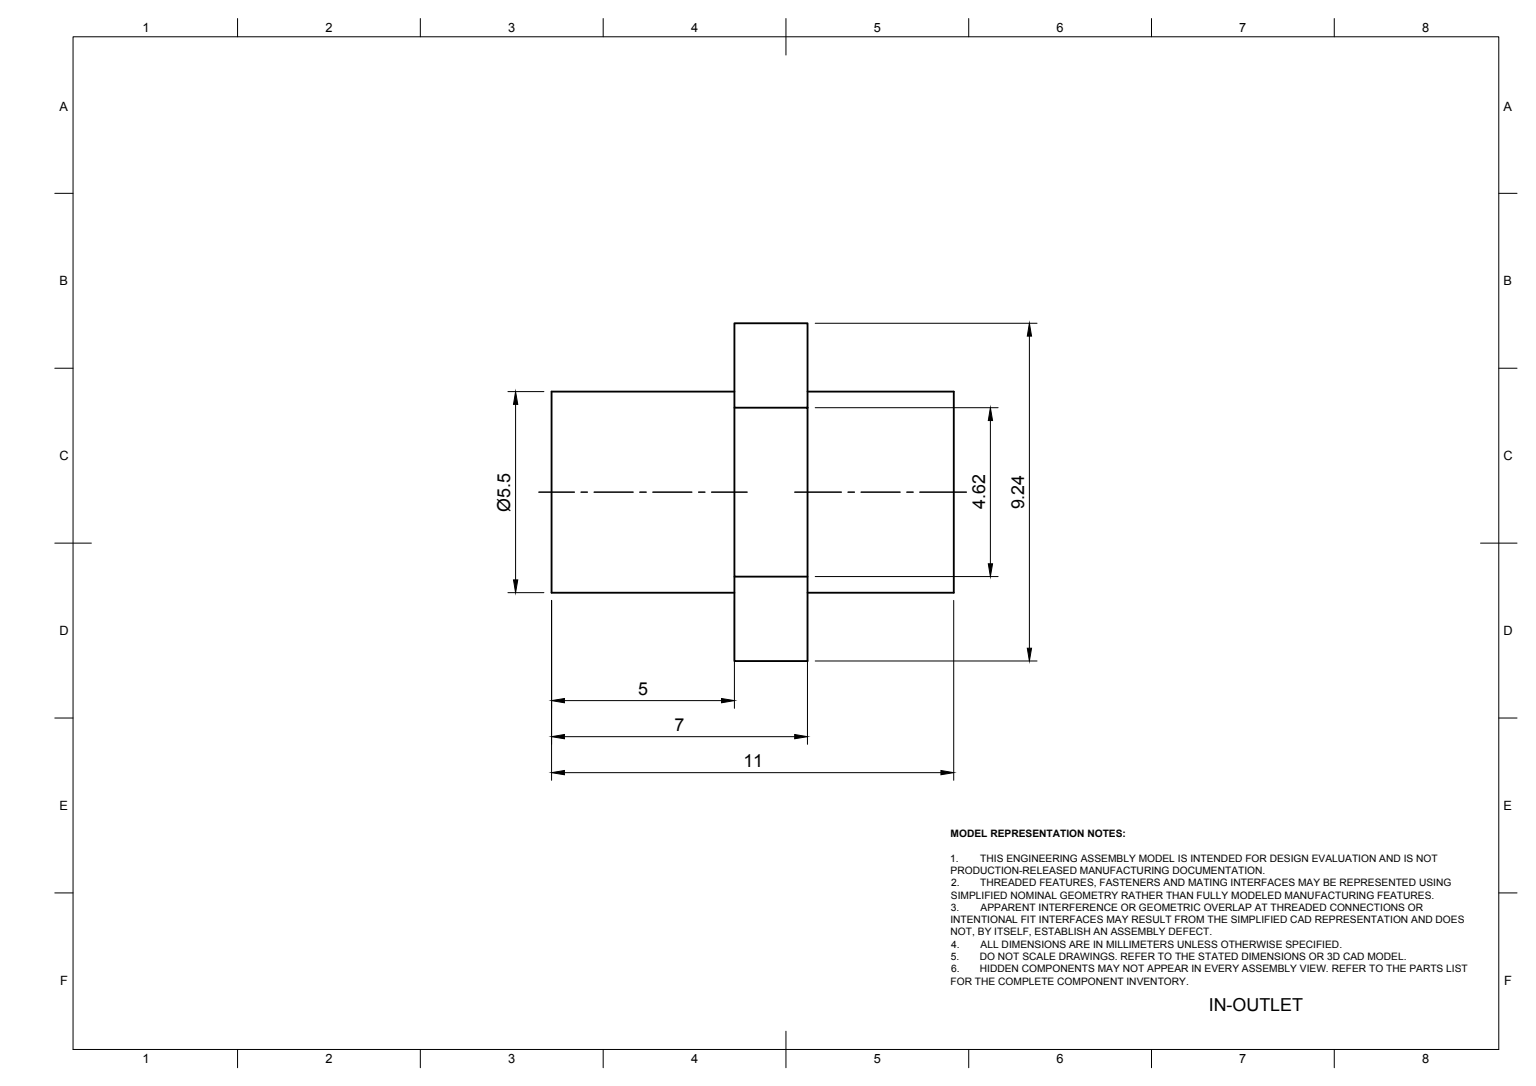
ISO-10303-21;
HEADER;
/* Generated by software containing ST-Developer
 * from STEP Tools, Inc. (www.steptools.com) 
 */

FILE_DESCRIPTION(
/* description */ (''),
/* implementation_level */ '2;1');

FILE_NAME(
/* name */ 'IN-OUTLET.step',
/* time_stamp */ '2026-10-06T01:16:10-07:00',
/* author */ (''),
/* organization */ (''),
/* preprocessor_version */ 'ST-DEVELOPER v20.2',
/* originating_system */ 'Autodesk Translation Framework v15.15.0.0',
/* authorisation */ '');

FILE_SCHEMA (('AUTOMOTIVE_DESIGN { 1 0 10303 214 3 1 1 }'));
ENDSEC;

DATA;
#10=MECHANICAL_DESIGN_GEOMETRIC_PRESENTATION_REPRESENTATION('',(#303,#304,#305),#17113);
#225=OPEN_SHELL('',(#5821,#5822));
#226=OPEN_SHELL('',(#5823,#5824));
#243=SHELL_BASED_SURFACE_MODEL('Body2',(#225));
#244=SHELL_BASED_SURFACE_MODEL('Body3',(#226));
#267=SHAPE_REPRESENTATION_RELATIONSHIP('SRR','None',#17189,#283);
#283=ADVANCED_BREP_SHAPE_REPRESENTATION('',(#333),#17096);
#303=STYLED_ITEM('',(#17298),#333);
#304=STYLED_ITEM('',(#17298),#243);
#305=STYLED_ITEM('',(#17298),#244);
#333=MANIFOLD_SOLID_BREP('Body1',#6019);
#410=CYLINDRICAL_SURFACE('',#6534,2.75);
#411=CYLINDRICAL_SURFACE('',#6536,2.75);
#412=CYLINDRICAL_SURFACE('',#6540,1.75);
#413=CYLINDRICAL_SURFACE('',#6543,2.475);
#414=CYLINDRICAL_SURFACE('',#6548,2.475);
#545=FACE_BOUND('',#1562,.T.);
#546=FACE_BOUND('',#1570,.T.);
#547=FACE_BOUND('',#1574,.T.);
#548=FACE_BOUND('',#1577,.T.);
#549=FACE_BOUND('',#1580,.T.);
#550=FACE_BOUND('',#1583,.T.);
#796=CIRCLE('',#6525,2.75);
#797=CIRCLE('',#6533,2.75);
#798=CIRCLE('',#6535,2.75);
#799=CIRCLE('',#6537,2.75);
#800=CIRCLE('',#6539,1.75);
#801=CIRCLE('',#6541,1.75);
#802=CIRCLE('',#6544,2.475);
#803=CIRCLE('',#6545,2.475);
#804=CIRCLE('',#6547,2.75);
#805=CIRCLE('',#6549,2.475);
#806=CIRCLE('',#6550,2.475);
#807=CIRCLE('',#6552,2.75);
#1160=FACE_OUTER_BOUND('',#1561,.T.);
#1161=FACE_OUTER_BOUND('',#1563,.T.);
#1162=FACE_OUTER_BOUND('',#1564,.T.);
#1163=FACE_OUTER_BOUND('',#1565,.T.);
#1164=FACE_OUTER_BOUND('',#1566,.T.);
#1165=FACE_OUTER_BOUND('',#1567,.T.);
#1166=FACE_OUTER_BOUND('',#1568,.T.);
#1167=FACE_OUTER_BOUND('',#1569,.T.);
#1168=FACE_OUTER_BOUND('',#1571,.T.);
#1169=FACE_OUTER_BOUND('',#1572,.T.);
#1170=FACE_OUTER_BOUND('',#1573,.T.);
#1171=FACE_OUTER_BOUND('',#1575,.T.);
#1172=FACE_OUTER_BOUND('',#1576,.T.);
#1173=FACE_OUTER_BOUND('',#1578,.T.);
#1174=FACE_OUTER_BOUND('',#1579,.T.);
#1175=FACE_OUTER_BOUND('',#1581,.T.);
#1176=FACE_OUTER_BOUND('',#1582,.T.);
#1561=EDGE_LOOP('',(#4622,#4623,#4624,#4625,#4626,#4627));
#1562=EDGE_LOOP('',(#4628));
#1563=EDGE_LOOP('',(#4629,#4630,#4631,#4632));
#1564=EDGE_LOOP('',(#4633,#4634,#4635,#4636));
#1565=EDGE_LOOP('',(#4637,#4638,#4639,#4640));
#1566=EDGE_LOOP('',(#4641,#4642,#4643,#4644));
#1567=EDGE_LOOP('',(#4645,#4646,#4647,#4648));
#1568=EDGE_LOOP('',(#4649,#4650,#4651,#4652));
#1569=EDGE_LOOP('',(#4653,#4654,#4655,#4656,#4657,#4658));
#1570=EDGE_LOOP('',(#4659));
#1571=EDGE_LOOP('',(#4660,#4661,#4662,#4663));
#1572=EDGE_LOOP('',(#4664,#4665,#4666,#4667));
#1573=EDGE_LOOP('',(#4668));
#1574=EDGE_LOOP('',(#4669));
#1575=EDGE_LOOP('',(#4670,#4671,#4672,#4673));
#1576=EDGE_LOOP('',(#4674));
#1577=EDGE_LOOP('',(#4675));
#1578=EDGE_LOOP('',(#4676,#4677,#4678,#4679));
#1579=EDGE_LOOP('',(#4680));
#1580=EDGE_LOOP('',(#4681));
#1581=EDGE_LOOP('',(#4682,#4683,#4684,#4685));
#1582=EDGE_LOOP('',(#4686));
#1583=EDGE_LOOP('',(#4687));
#2031=LINE('',#10370,#2392);
#2032=LINE('',#10372,#2393);
#2033=LINE('',#10374,#2394);
#2034=LINE('',#10376,#2395);
#2035=LINE('',#10378,#2396);
#2036=LINE('',#10379,#2397);
#2037=LINE('',#10384,#2398);
#2038=LINE('',#10386,#2399);
#2039=LINE('',#10387,#2400);
#2040=LINE('',#10390,#2401);
#2041=LINE('',#10391,#2402);
#2042=LINE('',#10394,#2403);
#2043=LINE('',#10395,#2404);
#2044=LINE('',#10398,#2405);
#2045=LINE('',#10399,#2406);
#2046=LINE('',#10402,#2407);
#2047=LINE('',#10403,#2408);
#2048=LINE('',#10405,#2409);
#2049=LINE('',#10411,#2410);
#2050=LINE('',#10416,#2411);
#2051=LINE('',#10422,#2412);
#2052=LINE('',#10429,#2413);
#2053=LINE('',#10438,#2414);
#2392=VECTOR('',#7781,4.618802153517);
#2393=VECTOR('',#7782,4.61880215351685);
#2394=VECTOR('',#7783,4.61880215351685);
#2395=VECTOR('',#7784,4.618802153517);
#2396=VECTOR('',#7785,4.61880215351685);
#2397=VECTOR('',#7786,4.61880215351685);
#2398=VECTOR('',#7791,2.);
#2399=VECTOR('',#7792,4.618802153517);
#2400=VECTOR('',#7793,2.);
#2401=VECTOR('',#7796,4.61880215351685);
#2402=VECTOR('',#7797,2.);
#2403=VECTOR('',#7800,4.61880215351685);
#2404=VECTOR('',#7801,2.);
#2405=VECTOR('',#7804,4.618802153517);
#2406=VECTOR('',#7805,2.);
#2407=VECTOR('',#7808,4.61880215351685);
#2408=VECTOR('',#7809,2.);
#2409=VECTOR('',#7812,4.61880215351685);
#2410=VECTOR('',#7819,2.75);
#2411=VECTOR('',#7826,2.75);
#2412=VECTOR('',#7833,1.75);
#2413=VECTOR('',#7842,2.475);
#2414=VECTOR('',#7853,2.475);
#2800=VERTEX_POINT('',#10368);
#2801=VERTEX_POINT('',#10369);
#2802=VERTEX_POINT('',#10371);
#2803=VERTEX_POINT('',#10373);
#2804=VERTEX_POINT('',#10375);
#2805=VERTEX_POINT('',#10377);
#2806=VERTEX_POINT('',#10380);
#2807=VERTEX_POINT('',#10383);
#2808=VERTEX_POINT('',#10385);
#2809=VERTEX_POINT('',#10389);
#2810=VERTEX_POINT('',#10393);
#2811=VERTEX_POINT('',#10397);
#2812=VERTEX_POINT('',#10401);
#2813=VERTEX_POINT('',#10407);
#2814=VERTEX_POINT('',#10410);
#2815=VERTEX_POINT('',#10414);
#2816=VERTEX_POINT('',#10418);
#2817=VERTEX_POINT('',#10421);
#2818=VERTEX_POINT('',#10426);
#2819=VERTEX_POINT('',#10428);
#2820=VERTEX_POINT('',#10432);
#2821=VERTEX_POINT('',#10435);
#2822=VERTEX_POINT('',#10437);
#2823=VERTEX_POINT('',#10441);
#3461=EDGE_CURVE('',#2800,#2801,#2031,.T.);
#3462=EDGE_CURVE('',#2802,#2800,#2032,.T.);
#3463=EDGE_CURVE('',#2803,#2802,#2033,.T.);
#3464=EDGE_CURVE('',#2804,#2803,#2034,.T.);
#3465=EDGE_CURVE('',#2805,#2804,#2035,.T.);
#3466=EDGE_CURVE('',#2801,#2805,#2036,.T.);
#3467=EDGE_CURVE('',#2806,#2806,#796,.T.);
#3468=EDGE_CURVE('',#2801,#2807,#2037,.T.);
#3469=EDGE_CURVE('',#2808,#2807,#2038,.T.);
#3470=EDGE_CURVE('',#2800,#2808,#2039,.T.);
#3471=EDGE_CURVE('',#2809,#2808,#2040,.T.);
#3472=EDGE_CURVE('',#2802,#2809,#2041,.T.);
#3473=EDGE_CURVE('',#2810,#2809,#2042,.T.);
#3474=EDGE_CURVE('',#2803,#2810,#2043,.T.);
#3475=EDGE_CURVE('',#2811,#2810,#2044,.T.);
#3476=EDGE_CURVE('',#2804,#2811,#2045,.T.);
#3477=EDGE_CURVE('',#2812,#2811,#2046,.T.);
#3478=EDGE_CURVE('',#2805,#2812,#2047,.T.);
#3479=EDGE_CURVE('',#2807,#2812,#2048,.T.);
#3480=EDGE_CURVE('',#2813,#2813,#797,.T.);
#3481=EDGE_CURVE('',#2806,#2814,#2049,.T.);
#3482=EDGE_CURVE('',#2814,#2814,#798,.T.);
#3483=EDGE_CURVE('',#2815,#2815,#799,.T.);
#3484=EDGE_CURVE('',#2815,#2813,#2050,.T.);
#3485=EDGE_CURVE('',#2816,#2816,#800,.T.);
#3486=EDGE_CURVE('',#2816,#2817,#2051,.T.);
#3487=EDGE_CURVE('',#2817,#2817,#801,.T.);
#3488=EDGE_CURVE('',#2818,#2818,#802,.T.);
#3489=EDGE_CURVE('',#2818,#2819,#2052,.T.);
#3490=EDGE_CURVE('',#2819,#2819,#803,.T.);
#3491=EDGE_CURVE('',#2820,#2820,#804,.T.);
#3492=EDGE_CURVE('',#2821,#2821,#805,.T.);
#3493=EDGE_CURVE('',#2821,#2822,#2053,.T.);
#3494=EDGE_CURVE('',#2822,#2822,#806,.T.);
#3495=EDGE_CURVE('',#2823,#2823,#807,.T.);
#4622=ORIENTED_EDGE('',*,*,#3461,.F.);
#4623=ORIENTED_EDGE('',*,*,#3462,.F.);
#4624=ORIENTED_EDGE('',*,*,#3463,.F.);
#4625=ORIENTED_EDGE('',*,*,#3464,.F.);
#4626=ORIENTED_EDGE('',*,*,#3465,.F.);
#4627=ORIENTED_EDGE('',*,*,#3466,.F.);
#4628=ORIENTED_EDGE('',*,*,#3467,.T.);
#4629=ORIENTED_EDGE('',*,*,#3461,.T.);
#4630=ORIENTED_EDGE('',*,*,#3468,.T.);
#4631=ORIENTED_EDGE('',*,*,#3469,.F.);
#4632=ORIENTED_EDGE('',*,*,#3470,.F.);
#4633=ORIENTED_EDGE('',*,*,#3462,.T.);
#4634=ORIENTED_EDGE('',*,*,#3470,.T.);
#4635=ORIENTED_EDGE('',*,*,#3471,.F.);
#4636=ORIENTED_EDGE('',*,*,#3472,.F.);
#4637=ORIENTED_EDGE('',*,*,#3463,.T.);
#4638=ORIENTED_EDGE('',*,*,#3472,.T.);
#4639=ORIENTED_EDGE('',*,*,#3473,.F.);
#4640=ORIENTED_EDGE('',*,*,#3474,.F.);
#4641=ORIENTED_EDGE('',*,*,#3464,.T.);
#4642=ORIENTED_EDGE('',*,*,#3474,.T.);
#4643=ORIENTED_EDGE('',*,*,#3475,.F.);
#4644=ORIENTED_EDGE('',*,*,#3476,.F.);
#4645=ORIENTED_EDGE('',*,*,#3465,.T.);
#4646=ORIENTED_EDGE('',*,*,#3476,.T.);
#4647=ORIENTED_EDGE('',*,*,#3477,.F.);
#4648=ORIENTED_EDGE('',*,*,#3478,.F.);
#4649=ORIENTED_EDGE('',*,*,#3466,.T.);
#4650=ORIENTED_EDGE('',*,*,#3478,.T.);
#4651=ORIENTED_EDGE('',*,*,#3479,.F.);
#4652=ORIENTED_EDGE('',*,*,#3468,.F.);
#4653=ORIENTED_EDGE('',*,*,#3469,.T.);
#4654=ORIENTED_EDGE('',*,*,#3479,.T.);
#4655=ORIENTED_EDGE('',*,*,#3477,.T.);
#4656=ORIENTED_EDGE('',*,*,#3475,.T.);
#4657=ORIENTED_EDGE('',*,*,#3473,.T.);
#4658=ORIENTED_EDGE('',*,*,#3471,.T.);
#4659=ORIENTED_EDGE('',*,*,#3480,.F.);
#4660=ORIENTED_EDGE('',*,*,#3467,.F.);
#4661=ORIENTED_EDGE('',*,*,#3481,.T.);
#4662=ORIENTED_EDGE('',*,*,#3482,.T.);
#4663=ORIENTED_EDGE('',*,*,#3481,.F.);
#4664=ORIENTED_EDGE('',*,*,#3483,.F.);
#4665=ORIENTED_EDGE('',*,*,#3484,.T.);
#4666=ORIENTED_EDGE('',*,*,#3480,.T.);
#4667=ORIENTED_EDGE('',*,*,#3484,.F.);
#4668=ORIENTED_EDGE('',*,*,#3482,.F.);
#4669=ORIENTED_EDGE('',*,*,#3485,.T.);
#4670=ORIENTED_EDGE('',*,*,#3485,.F.);
#4671=ORIENTED_EDGE('',*,*,#3486,.T.);
#4672=ORIENTED_EDGE('',*,*,#3487,.T.);
#4673=ORIENTED_EDGE('',*,*,#3486,.F.);
#4674=ORIENTED_EDGE('',*,*,#3483,.T.);
#4675=ORIENTED_EDGE('',*,*,#3487,.F.);
#4676=ORIENTED_EDGE('',*,*,#3488,.F.);
#4677=ORIENTED_EDGE('',*,*,#3489,.T.);
#4678=ORIENTED_EDGE('',*,*,#3490,.T.);
#4679=ORIENTED_EDGE('',*,*,#3489,.F.);
#4680=ORIENTED_EDGE('',*,*,#3491,.F.);
#4681=ORIENTED_EDGE('',*,*,#3490,.F.);
#4682=ORIENTED_EDGE('',*,*,#3492,.F.);
#4683=ORIENTED_EDGE('',*,*,#3493,.T.);
#4684=ORIENTED_EDGE('',*,*,#3494,.T.);
#4685=ORIENTED_EDGE('',*,*,#3493,.F.);
#4686=ORIENTED_EDGE('',*,*,#3495,.F.);
#4687=ORIENTED_EDGE('',*,*,#3494,.F.);
#5559=PLANE('',#6524);
#5560=PLANE('',#6526);
#5561=PLANE('',#6527);
#5562=PLANE('',#6528);
#5563=PLANE('',#6529);
#5564=PLANE('',#6530);
#5565=PLANE('',#6531);
#5566=PLANE('',#6532);
#5567=PLANE('',#6538);
#5568=PLANE('',#6542);
#5569=PLANE('',#6546);
#5570=PLANE('',#6551);
#5808=ADVANCED_FACE('',(#1160,#545),#5559,.F.);
#5809=ADVANCED_FACE('',(#1161),#5560,.T.);
#5810=ADVANCED_FACE('',(#1162),#5561,.T.);
#5811=ADVANCED_FACE('',(#1163),#5562,.T.);
#5812=ADVANCED_FACE('',(#1164),#5563,.T.);
#5813=ADVANCED_FACE('',(#1165),#5564,.T.);
#5814=ADVANCED_FACE('',(#1166),#5565,.T.);
#5815=ADVANCED_FACE('',(#1167,#546),#5566,.T.);
#5816=ADVANCED_FACE('',(#1168),#410,.T.);
#5817=ADVANCED_FACE('',(#1169),#411,.T.);
#5818=ADVANCED_FACE('',(#1170,#547),#5567,.F.);
#5819=ADVANCED_FACE('',(#1171),#412,.F.);
#5820=ADVANCED_FACE('',(#1172,#548),#5568,.T.);
#5821=ADVANCED_FACE('',(#1173),#413,.T.);
#5822=ADVANCED_FACE('',(#1174,#549),#5569,.T.);
#5823=ADVANCED_FACE('',(#1175),#414,.T.);
#5824=ADVANCED_FACE('',(#1176,#550),#5570,.T.);
#6019=CLOSED_SHELL('',(#5808,#5809,#5810,#5811,#5812,#5813,#5814,#5815,
#5816,#5817,#5818,#5819,#5820));
#6523=AXIS2_PLACEMENT_3D('',#10366,#7777,#7778);
#6524=AXIS2_PLACEMENT_3D('',#10367,#7779,#7780);
#6525=AXIS2_PLACEMENT_3D('',#10381,#7787,#7788);
#6526=AXIS2_PLACEMENT_3D('',#10382,#7789,#7790);
#6527=AXIS2_PLACEMENT_3D('',#10388,#7794,#7795);
#6528=AXIS2_PLACEMENT_3D('',#10392,#7798,#7799);
#6529=AXIS2_PLACEMENT_3D('',#10396,#7802,#7803);
#6530=AXIS2_PLACEMENT_3D('',#10400,#7806,#7807);
#6531=AXIS2_PLACEMENT_3D('',#10404,#7810,#7811);
#6532=AXIS2_PLACEMENT_3D('',#10406,#7813,#7814);
#6533=AXIS2_PLACEMENT_3D('',#10408,#7815,#7816);
#6534=AXIS2_PLACEMENT_3D('',#10409,#7817,#7818);
#6535=AXIS2_PLACEMENT_3D('',#10412,#7820,#7821);
#6536=AXIS2_PLACEMENT_3D('',#10413,#7822,#7823);
#6537=AXIS2_PLACEMENT_3D('',#10415,#7824,#7825);
#6538=AXIS2_PLACEMENT_3D('',#10417,#7827,#7828);
#6539=AXIS2_PLACEMENT_3D('',#10419,#7829,#7830);
#6540=AXIS2_PLACEMENT_3D('',#10420,#7831,#7832);
#6541=AXIS2_PLACEMENT_3D('',#10423,#7834,#7835);
#6542=AXIS2_PLACEMENT_3D('',#10424,#7836,#7837);
#6543=AXIS2_PLACEMENT_3D('',#10425,#7838,#7839);
#6544=AXIS2_PLACEMENT_3D('',#10427,#7840,#7841);
#6545=AXIS2_PLACEMENT_3D('',#10430,#7843,#7844);
#6546=AXIS2_PLACEMENT_3D('',#10431,#7845,#7846);
#6547=AXIS2_PLACEMENT_3D('',#10433,#7847,#7848);
#6548=AXIS2_PLACEMENT_3D('',#10434,#7849,#7850);
#6549=AXIS2_PLACEMENT_3D('',#10436,#7851,#7852);
#6550=AXIS2_PLACEMENT_3D('',#10439,#7854,#7855);
#6551=AXIS2_PLACEMENT_3D('',#10440,#7856,#7857);
#6552=AXIS2_PLACEMENT_3D('',#10442,#7858,#7859);
#7777=DIRECTION('axis',(0.,0.,1.));
#7778=DIRECTION('refdir',(1.,0.,0.));
#7779=DIRECTION('center_axis',(0.,0.,1.));
#7780=DIRECTION('ref_axis',(1.,0.,0.));
#7781=DIRECTION('',(1.,0.,0.));
#7782=DIRECTION('',(0.500000000000017,-0.866025403784429,0.));
#7783=DIRECTION('',(-0.500000000000017,-0.866025403784429,0.));
#7784=DIRECTION('',(-1.,0.,0.));
#7785=DIRECTION('',(-0.500000000000017,0.866025403784429,0.));
#7786=DIRECTION('',(0.500000000000017,0.866025403784429,0.));
#7787=DIRECTION('center_axis',(0.,0.,1.));
#7788=DIRECTION('ref_axis',(1.,0.,0.));
#7789=DIRECTION('center_axis',(0.,-1.,0.));
#7790=DIRECTION('ref_axis',(1.,0.,0.));
#7791=DIRECTION('',(0.,0.,1.));
#7792=DIRECTION('',(1.,0.,0.));
#7793=DIRECTION('',(0.,0.,1.));
#7794=DIRECTION('center_axis',(-0.866025403784429,-0.500000000000017,0.));
#7795=DIRECTION('ref_axis',(0.500000000000017,-0.866025403784429,0.));
#7796=DIRECTION('',(0.500000000000017,-0.866025403784429,0.));
#7797=DIRECTION('',(0.,0.,1.));
#7798=DIRECTION('center_axis',(-0.866025403784429,0.500000000000017,0.));
#7799=DIRECTION('ref_axis',(-0.500000000000017,-0.866025403784429,0.));
#7800=DIRECTION('',(-0.500000000000017,-0.866025403784429,0.));
#7801=DIRECTION('',(0.,0.,1.));
#7802=DIRECTION('center_axis',(0.,1.,0.));
#7803=DIRECTION('ref_axis',(-1.,0.,0.));
#7804=DIRECTION('',(-1.,0.,0.));
#7805=DIRECTION('',(0.,0.,1.));
#7806=DIRECTION('center_axis',(0.866025403784429,0.500000000000017,0.));
#7807=DIRECTION('ref_axis',(-0.500000000000017,0.866025403784429,0.));
#7808=DIRECTION('',(-0.500000000000017,0.866025403784429,0.));
#7809=DIRECTION('',(0.,0.,1.));
#7810=DIRECTION('center_axis',(0.866025403784429,-0.500000000000017,0.));
#7811=DIRECTION('ref_axis',(0.500000000000017,0.866025403784429,0.));
#7812=DIRECTION('',(0.500000000000017,0.866025403784429,0.));
#7813=DIRECTION('center_axis',(0.,0.,1.));
#7814=DIRECTION('ref_axis',(1.,0.,0.));
#7815=DIRECTION('center_axis',(0.,0.,1.));
#7816=DIRECTION('ref_axis',(1.,0.,0.));
#7817=DIRECTION('center_axis',(0.,0.,1.));
#7818=DIRECTION('ref_axis',(1.,0.,0.));
#7819=DIRECTION('',(0.,0.,-1.));
#7820=DIRECTION('center_axis',(0.,0.,1.));
#7821=DIRECTION('ref_axis',(1.,0.,0.));
#7822=DIRECTION('center_axis',(0.,0.,1.));
#7823=DIRECTION('ref_axis',(1.,0.,0.));
#7824=DIRECTION('center_axis',(0.,0.,1.));
#7825=DIRECTION('ref_axis',(1.,0.,0.));
#7826=DIRECTION('',(0.,0.,-1.));
#7827=DIRECTION('center_axis',(0.,0.,1.));
#7828=DIRECTION('ref_axis',(1.,0.,0.));
#7829=DIRECTION('center_axis',(0.,0.,1.));
#7830=DIRECTION('ref_axis',(1.,0.,0.));
#7831=DIRECTION('center_axis',(0.,0.,1.));
#7832=DIRECTION('ref_axis',(1.,0.,0.));
#7833=DIRECTION('',(0.,0.,1.));
#7834=DIRECTION('center_axis',(0.,0.,1.));
#7835=DIRECTION('ref_axis',(1.,0.,0.));
#7836=DIRECTION('center_axis',(0.,0.,1.));
#7837=DIRECTION('ref_axis',(1.,0.,0.));
#7838=DIRECTION('center_axis',(0.,0.,1.));
#7839=DIRECTION('ref_axis',(1.,0.,0.));
#7840=DIRECTION('center_axis',(0.,0.,1.));
#7841=DIRECTION('ref_axis',(-1.,0.,0.));
#7842=DIRECTION('',(0.,0.,-1.));
#7843=DIRECTION('center_axis',(0.,0.,1.));
#7844=DIRECTION('ref_axis',(-1.,0.,0.));
#7845=DIRECTION('center_axis',(0.,0.,1.));
#7846=DIRECTION('ref_axis',(1.,0.,0.));
#7847=DIRECTION('center_axis',(0.,0.,-1.));
#7848=DIRECTION('ref_axis',(-1.,0.,0.));
#7849=DIRECTION('center_axis',(0.,0.,-1.));
#7850=DIRECTION('ref_axis',(-1.,0.,0.));
#7851=DIRECTION('center_axis',(0.,0.,-1.));
#7852=DIRECTION('ref_axis',(1.,0.,0.));
#7853=DIRECTION('',(0.,0.,1.));
#7854=DIRECTION('center_axis',(0.,0.,-1.));
#7855=DIRECTION('ref_axis',(1.,0.,0.));
#7856=DIRECTION('center_axis',(0.,0.,-1.));
#7857=DIRECTION('ref_axis',(-1.,0.,0.));
#7858=DIRECTION('center_axis',(0.,0.,1.));
#7859=DIRECTION('ref_axis',(1.,0.,0.));
#10366=CARTESIAN_POINT('',(0.,0.,0.));
#10367=CARTESIAN_POINT('Origin',(0.,0.,-1.));
#10368=CARTESIAN_POINT('',(-2.309401076759,-4.,-1.));
#10369=CARTESIAN_POINT('',(2.309401076759,-4.,-1.));
#10370=CARTESIAN_POINT('',(-2.309401076759,-4.,-1.));
#10371=CARTESIAN_POINT('',(-4.618802153517,0.,-1.));
#10372=CARTESIAN_POINT('',(-4.618802153517,0.,-1.));
#10373=CARTESIAN_POINT('',(-2.309401076759,4.,-1.));
#10374=CARTESIAN_POINT('',(-2.309401076759,4.,-1.));
#10375=CARTESIAN_POINT('',(2.309401076759,4.,-1.));
#10376=CARTESIAN_POINT('',(2.309401076759,4.,-1.));
#10377=CARTESIAN_POINT('',(4.618802153517,0.,-1.));
#10378=CARTESIAN_POINT('',(4.618802153517,0.,-1.));
#10379=CARTESIAN_POINT('',(2.309401076759,-4.,-1.));
#10380=CARTESIAN_POINT('',(-2.75,0.,-1.));
#10381=CARTESIAN_POINT('Origin',(0.,0.,-1.));
#10382=CARTESIAN_POINT('Origin',(-2.309401076759,-4.,-1.));
#10383=CARTESIAN_POINT('',(2.309401076759,-4.,1.));
#10384=CARTESIAN_POINT('',(2.309401076759,-4.,-1.));
#10385=CARTESIAN_POINT('',(-2.309401076759,-4.,1.));
#10386=CARTESIAN_POINT('',(-2.309401076759,-4.,1.));
#10387=CARTESIAN_POINT('',(-2.309401076759,-4.,-1.));
#10388=CARTESIAN_POINT('Origin',(-4.618802153517,0.,-1.));
#10389=CARTESIAN_POINT('',(-4.618802153517,0.,1.));
#10390=CARTESIAN_POINT('',(-4.618802153517,0.,1.));
#10391=CARTESIAN_POINT('',(-4.618802153517,0.,-1.));
#10392=CARTESIAN_POINT('Origin',(-2.309401076759,4.,-1.));
#10393=CARTESIAN_POINT('',(-2.309401076759,4.,1.));
#10394=CARTESIAN_POINT('',(-2.309401076759,4.,1.));
#10395=CARTESIAN_POINT('',(-2.309401076759,4.,-1.));
#10396=CARTESIAN_POINT('Origin',(2.309401076759,4.,-1.));
#10397=CARTESIAN_POINT('',(2.309401076759,4.,1.));
#10398=CARTESIAN_POINT('',(2.309401076759,4.,1.));
#10399=CARTESIAN_POINT('',(2.309401076759,4.,-1.));
#10400=CARTESIAN_POINT('Origin',(4.618802153517,0.,-1.));
#10401=CARTESIAN_POINT('',(4.618802153517,0.,1.));
#10402=CARTESIAN_POINT('',(4.618802153517,0.,1.));
#10403=CARTESIAN_POINT('',(4.618802153517,0.,-1.));
#10404=CARTESIAN_POINT('Origin',(2.309401076759,-4.,-1.));
#10405=CARTESIAN_POINT('',(2.309401076759,-4.,1.));
#10406=CARTESIAN_POINT('Origin',(0.,0.,1.));
#10407=CARTESIAN_POINT('',(-2.75,-3.36777869765522E-16,1.));
#10408=CARTESIAN_POINT('Origin',(0.,0.,1.));
#10409=CARTESIAN_POINT('Origin',(0.,0.,-5.));
#10410=CARTESIAN_POINT('',(-2.75,0.,-5.));
#10411=CARTESIAN_POINT('',(-2.75,-3.36777869765522E-16,-5.));
#10412=CARTESIAN_POINT('Origin',(0.,0.,-5.));
#10413=CARTESIAN_POINT('Origin',(0.,0.,-5.));
#10414=CARTESIAN_POINT('',(-2.75,-3.36777869765522E-16,6.));
#10415=CARTESIAN_POINT('Origin',(0.,0.,6.));
#10416=CARTESIAN_POINT('',(-2.75,-3.36777869765522E-16,-5.));
#10417=CARTESIAN_POINT('Origin',(0.,0.,-5.));
#10418=CARTESIAN_POINT('',(-1.75,0.,-5.));
#10419=CARTESIAN_POINT('Origin',(0.,0.,-5.));
#10420=CARTESIAN_POINT('Origin',(0.,0.,6.));
#10421=CARTESIAN_POINT('',(-1.75,0.,6.));
#10422=CARTESIAN_POINT('',(-1.75,-2.14313189850787E-16,6.));
#10423=CARTESIAN_POINT('Origin',(0.,0.,6.));
#10424=CARTESIAN_POINT('Origin',(0.,0.,6.));
#10425=CARTESIAN_POINT('Origin',(0.,0.,6.));
#10426=CARTESIAN_POINT('',(-2.475,-3.0310008278897E-16,6.));
#10427=CARTESIAN_POINT('Origin',(0.,0.,6.));
#10428=CARTESIAN_POINT('',(-2.475,-3.0310008278897E-16,1.));
#10429=CARTESIAN_POINT('',(-2.475,-3.0310008278897E-16,6.));
#10430=CARTESIAN_POINT('Origin',(0.,0.,1.));
#10431=CARTESIAN_POINT('Origin',(0.,0.,1.));
#10432=CARTESIAN_POINT('',(2.75,0.,1.));
#10433=CARTESIAN_POINT('Origin',(0.,0.,1.));
#10434=CARTESIAN_POINT('Origin',(0.,0.,-5.));
#10435=CARTESIAN_POINT('',(2.475,-3.0310008278897E-16,-5.));
#10436=CARTESIAN_POINT('Origin',(0.,0.,-5.));
#10437=CARTESIAN_POINT('',(2.475,-3.0310008278897E-16,-1.));
#10438=CARTESIAN_POINT('',(2.475,-3.0310008278897E-16,-5.));
#10439=CARTESIAN_POINT('Origin',(0.,0.,-1.));
#10440=CARTESIAN_POINT('Origin',(0.,0.,-1.));
#10441=CARTESIAN_POINT('',(-2.75,0.,-1.));
#10442=CARTESIAN_POINT('Origin',(0.,0.,-1.));
#17073=UNCERTAINTY_MEASURE_WITH_UNIT(LENGTH_MEASURE(0.01),#17114,
'DISTANCE_ACCURACY_VALUE',
'Maximum model space distance between geometric entities at asserted c
onnectivities');
#17090=UNCERTAINTY_MEASURE_WITH_UNIT(LENGTH_MEASURE(0.01),#17114,
'DISTANCE_ACCURACY_VALUE',
'Maximum model space distance between geometric entities at asserted c
onnectivities');
#17096=(
GEOMETRIC_REPRESENTATION_CONTEXT(3)
GLOBAL_UNCERTAINTY_ASSIGNED_CONTEXT((#17073))
GLOBAL_UNIT_ASSIGNED_CONTEXT((#17114,#17116,#17117))
REPRESENTATION_CONTEXT('','3D')
);
#17113=(
GEOMETRIC_REPRESENTATION_CONTEXT(3)
GLOBAL_UNCERTAINTY_ASSIGNED_CONTEXT((#17090))
GLOBAL_UNIT_ASSIGNED_CONTEXT((#17114,#17116,#17117))
REPRESENTATION_CONTEXT('','3D')
);
#17114=(
LENGTH_UNIT()
NAMED_UNIT(*)
SI_UNIT(.MILLI.,.METRE.)
);
#17116=(
NAMED_UNIT(*)
PLANE_ANGLE_UNIT()
SI_UNIT($,.RADIAN.)
);
#17117=(
NAMED_UNIT(*)
SI_UNIT($,.STERADIAN.)
SOLID_ANGLE_UNIT()
);
#17123=SHAPE_DEFINITION_REPRESENTATION(#17145,#17189);
#17145=PRODUCT_DEFINITION_SHAPE('',$,#17212);
#17189=SHAPE_REPRESENTATION('',(#6523,#243,#244),#17096);
#17206=PRODUCT_DEFINITION_CONTEXT('part definition',#17274,'design');
#17212=PRODUCT_DEFINITION('IN-OUTLET','IN-OUTLET',#17234,#17206);
#17234=PRODUCT_DEFINITION_FORMATION('',$,#17281);
#17274=APPLICATION_CONTEXT(
'Core Data for Automotive Mechanical Design Process');
#17275=PRODUCT_CONTEXT('part definition',#17274,'mechanical');
#17281=PRODUCT('IN-OUTLET','IN-OUTLET','NOT SPECIFIED',(#17275));
#17298=PRESENTATION_STYLE_ASSIGNMENT((#17299));
#17299=SURFACE_STYLE_USAGE(.BOTH.,#17300);
#17300=SURFACE_SIDE_STYLE('',(#17301));
#17301=SURFACE_STYLE_FILL_AREA(#17302);
#17302=FILL_AREA_STYLE('Steel - Satin',(#17303));
#17303=FILL_AREA_STYLE_COLOUR('Steel - Satin',#17304);
#17304=COLOUR_RGB('Steel - Satin', 0.09019608, 0.27058824, 0.51372549);
ENDSEC;
END-ISO-10303-21;
